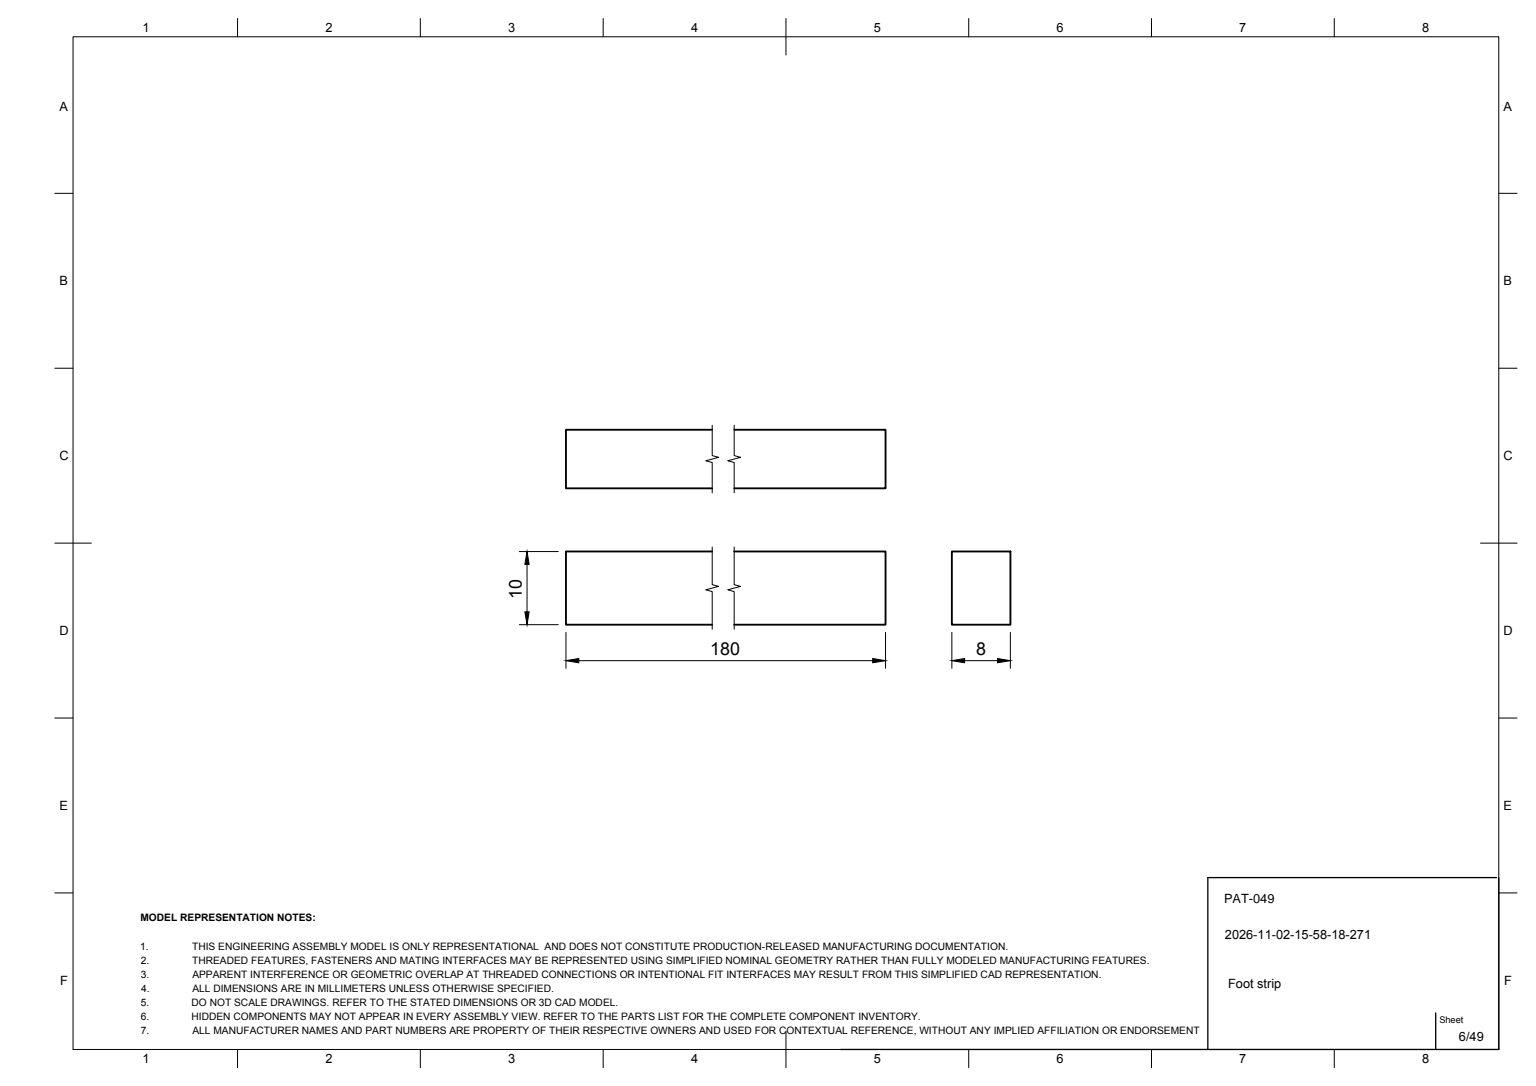
ISO-10303-21;
HEADER;
/* Generated by software containing ST-Developer
 * from STEP Tools, Inc. (www.steptools.com) 
 */

FILE_DESCRIPTION(
/* description */ ('Hand drill press frame (manual)'),
/* implementation_level */ '2;1');

FILE_NAME(
/* name */ 'Foot strip.step',
/* time_stamp */ '2026-10-28T03:25:28-07:00',
/* author */ (''),
/* organization */ (''),
/* preprocessor_version */ 'ST-DEVELOPER v20.2',
/* originating_system */ 'Autodesk Translation Framework v15.17.0.0',
/* authorisation */ '');

FILE_SCHEMA (('AUTOMOTIVE_DESIGN { 1 0 10303 214 3 1 1 }'));
ENDSEC;

DATA;
#10=MECHANICAL_DESIGN_GEOMETRIC_PRESENTATION_REPRESENTATION('',(#620),#33299);
#530=SHAPE_REPRESENTATION_RELATIONSHIP('SRR','None',#33489,#575);
#575=ADVANCED_BREP_SHAPE_REPRESENTATION('',(#672),#33251);
#620=STYLED_ITEM('',(#33800),#672);
#672=MANIFOLD_SOLID_BREP('Body1',#12638);
#893=PLANE('',#13216);
#894=PLANE('',#13217);
#895=PLANE('',#13218);
#896=PLANE('',#13219);
#897=PLANE('',#13220);
#898=PLANE('',#13221);
#1351=FACE_OUTER_BOUND('',#2052,.T.);
#1352=FACE_OUTER_BOUND('',#2053,.T.);
#1353=FACE_OUTER_BOUND('',#2054,.T.);
#1354=FACE_OUTER_BOUND('',#2055,.T.);
#1355=FACE_OUTER_BOUND('',#2056,.T.);
#1356=FACE_OUTER_BOUND('',#2057,.T.);
#2052=EDGE_LOOP('',(#8481,#8482,#8483,#8484));
#2053=EDGE_LOOP('',(#8485,#8486,#8487,#8488));
#2054=EDGE_LOOP('',(#8489,#8490,#8491,#8492));
#2055=EDGE_LOOP('',(#8493,#8494,#8495,#8496));
#2056=EDGE_LOOP('',(#8497,#8498,#8499,#8500));
#2057=EDGE_LOOP('',(#8501,#8502,#8503,#8504));
#2902=LINE('',#17959,#4067);
#2903=LINE('',#17961,#4068);
#2904=LINE('',#17963,#4069);
#2905=LINE('',#17964,#4070);
#2906=LINE('',#17967,#4071);
#2907=LINE('',#17969,#4072);
#2908=LINE('',#17970,#4073);
#2909=LINE('',#17973,#4074);
#2910=LINE('',#17975,#4075);
#2911=LINE('',#17976,#4076);
#2912=LINE('',#17978,#4077);
#2913=LINE('',#17979,#4078);
#4067=VECTOR('',#14443,1.);
#4068=VECTOR('',#14444,1.);
#4069=VECTOR('',#14445,1.);
#4070=VECTOR('',#14446,1.);
#4071=VECTOR('',#14449,1.);
#4072=VECTOR('',#14450,1.);
#4073=VECTOR('',#14451,1.);
#4074=VECTOR('',#14454,1.);
#4075=VECTOR('',#14455,1.);
#4076=VECTOR('',#14456,1.);
#4077=VECTOR('',#14459,1.);
#4078=VECTOR('',#14460,1.);
#5633=VERTEX_POINT('',#17957);
#5634=VERTEX_POINT('',#17958);
#5635=VERTEX_POINT('',#17960);
#5636=VERTEX_POINT('',#17962);
#5637=VERTEX_POINT('',#17966);
#5638=VERTEX_POINT('',#17968);
#5639=VERTEX_POINT('',#17972);
#5640=VERTEX_POINT('',#17974);
#6769=EDGE_CURVE('',#5633,#5634,#2902,.T.);
#6770=EDGE_CURVE('',#5634,#5635,#2903,.T.);
#6771=EDGE_CURVE('',#5636,#5635,#2904,.T.);
#6772=EDGE_CURVE('',#5633,#5636,#2905,.T.);
#6773=EDGE_CURVE('',#5637,#5633,#2906,.T.);
#6774=EDGE_CURVE('',#5638,#5636,#2907,.T.);
#6775=EDGE_CURVE('',#5637,#5638,#2908,.T.);
#6776=EDGE_CURVE('',#5639,#5637,#2909,.T.);
#6777=EDGE_CURVE('',#5640,#5638,#2910,.T.);
#6778=EDGE_CURVE('',#5639,#5640,#2911,.T.);
#6779=EDGE_CURVE('',#5634,#5639,#2912,.T.);
#6780=EDGE_CURVE('',#5635,#5640,#2913,.T.);
#8481=ORIENTED_EDGE('',*,*,#6769,.T.);
#8482=ORIENTED_EDGE('',*,*,#6770,.T.);
#8483=ORIENTED_EDGE('',*,*,#6771,.F.);
#8484=ORIENTED_EDGE('',*,*,#6772,.F.);
#8485=ORIENTED_EDGE('',*,*,#6773,.T.);
#8486=ORIENTED_EDGE('',*,*,#6772,.T.);
#8487=ORIENTED_EDGE('',*,*,#6774,.F.);
#8488=ORIENTED_EDGE('',*,*,#6775,.F.);
#8489=ORIENTED_EDGE('',*,*,#6776,.T.);
#8490=ORIENTED_EDGE('',*,*,#6775,.T.);
#8491=ORIENTED_EDGE('',*,*,#6777,.F.);
#8492=ORIENTED_EDGE('',*,*,#6778,.F.);
#8493=ORIENTED_EDGE('',*,*,#6779,.T.);
#8494=ORIENTED_EDGE('',*,*,#6778,.T.);
#8495=ORIENTED_EDGE('',*,*,#6780,.F.);
#8496=ORIENTED_EDGE('',*,*,#6770,.F.);
#8497=ORIENTED_EDGE('',*,*,#6780,.T.);
#8498=ORIENTED_EDGE('',*,*,#6777,.T.);
#8499=ORIENTED_EDGE('',*,*,#6774,.T.);
#8500=ORIENTED_EDGE('',*,*,#6771,.T.);
#8501=ORIENTED_EDGE('',*,*,#6779,.F.);
#8502=ORIENTED_EDGE('',*,*,#6769,.F.);
#8503=ORIENTED_EDGE('',*,*,#6773,.F.);
#8504=ORIENTED_EDGE('',*,*,#6776,.F.);
#11960=ADVANCED_FACE('',(#1351),#893,.T.);
#11961=ADVANCED_FACE('',(#1352),#894,.T.);
#11962=ADVANCED_FACE('',(#1353),#895,.T.);
#11963=ADVANCED_FACE('',(#1354),#896,.T.);
#11964=ADVANCED_FACE('',(#1355),#897,.T.);
#11965=ADVANCED_FACE('',(#1356),#898,.F.);
#12638=CLOSED_SHELL('',(#11960,#11961,#11962,#11963,#11964,#11965));
#13215=AXIS2_PLACEMENT_3D('',#17955,#14439,#14440);
#13216=AXIS2_PLACEMENT_3D('',#17956,#14441,#14442);
#13217=AXIS2_PLACEMENT_3D('',#17965,#14447,#14448);
#13218=AXIS2_PLACEMENT_3D('',#17971,#14452,#14453);
#13219=AXIS2_PLACEMENT_3D('',#17977,#14457,#14458);
#13220=AXIS2_PLACEMENT_3D('',#17980,#14461,#14462);
#13221=AXIS2_PLACEMENT_3D('',#17981,#14463,#14464);
#14439=DIRECTION('axis',(0.,0.,1.));
#14440=DIRECTION('refdir',(1.,0.,0.));
#14441=DIRECTION('center_axis',(0.,1.,0.));
#14442=DIRECTION('ref_axis',(-1.,0.,0.));
#14443=DIRECTION('',(-1.,0.,0.));
#14444=DIRECTION('',(0.,0.,1.));
#14445=DIRECTION('',(-1.,0.,0.));
#14446=DIRECTION('',(0.,0.,1.));
#14447=DIRECTION('center_axis',(1.,0.,0.));
#14448=DIRECTION('ref_axis',(0.,1.,0.));
#14449=DIRECTION('',(0.,1.,0.));
#14450=DIRECTION('',(0.,1.,0.));
#14451=DIRECTION('',(0.,0.,1.));
#14452=DIRECTION('center_axis',(0.,-1.,0.));
#14453=DIRECTION('ref_axis',(1.,0.,0.));
#14454=DIRECTION('',(1.,0.,0.));
#14455=DIRECTION('',(1.,0.,0.));
#14456=DIRECTION('',(0.,0.,1.));
#14457=DIRECTION('center_axis',(-1.,0.,0.));
#14458=DIRECTION('ref_axis',(0.,-1.,0.));
#14459=DIRECTION('',(0.,-1.,0.));
#14460=DIRECTION('',(0.,-1.,0.));
#14461=DIRECTION('center_axis',(0.,0.,1.));
#14462=DIRECTION('ref_axis',(1.,0.,0.));
#14463=DIRECTION('center_axis',(0.,0.,1.));
#14464=DIRECTION('ref_axis',(1.,0.,0.));
#17955=CARTESIAN_POINT('',(0.,0.,0.));
#17956=CARTESIAN_POINT('Origin',(-7.,9.,-0.8));
#17957=CARTESIAN_POINT('',(-7.,9.,-0.8));
#17958=CARTESIAN_POINT('',(-8.,9.,-0.8));
#17959=CARTESIAN_POINT('',(-7.,9.,-0.8));
#17960=CARTESIAN_POINT('',(-8.,9.,0.));
#17961=CARTESIAN_POINT('',(-8.,9.,-0.8));
#17962=CARTESIAN_POINT('',(-7.,9.,0.));
#17963=CARTESIAN_POINT('',(-7.,9.,0.));
#17964=CARTESIAN_POINT('',(-7.,9.,-0.8));
#17965=CARTESIAN_POINT('Origin',(-7.,-9.,-0.8));
#17966=CARTESIAN_POINT('',(-7.,-9.,-0.8));
#17967=CARTESIAN_POINT('',(-7.,-9.,-0.8));
#17968=CARTESIAN_POINT('',(-7.,-9.,0.));
#17969=CARTESIAN_POINT('',(-7.,-9.,0.));
#17970=CARTESIAN_POINT('',(-7.,-9.,-0.8));
#17971=CARTESIAN_POINT('Origin',(-8.,-9.,-0.8));
#17972=CARTESIAN_POINT('',(-8.,-9.,-0.8));
#17973=CARTESIAN_POINT('',(-8.,-9.,-0.8));
#17974=CARTESIAN_POINT('',(-8.,-9.,0.));
#17975=CARTESIAN_POINT('',(-8.,-9.,0.));
#17976=CARTESIAN_POINT('',(-8.,-9.,-0.8));
#17977=CARTESIAN_POINT('Origin',(-8.,9.,-0.8));
#17978=CARTESIAN_POINT('',(-8.,9.,-0.8));
#17979=CARTESIAN_POINT('',(-8.,9.,0.));
#17980=CARTESIAN_POINT('Origin',(-7.5,0.,0.));
#17981=CARTESIAN_POINT('Origin',(-7.5,0.,-0.8));
#33199=UNCERTAINTY_MEASURE_WITH_UNIT(LENGTH_MEASURE(0.001),#33300,
'DISTANCE_ACCURACY_VALUE',
'Maximum model space distance between geometric entities at asserted c
onnectivities');
#33247=UNCERTAINTY_MEASURE_WITH_UNIT(LENGTH_MEASURE(0.001),#33300,
'DISTANCE_ACCURACY_VALUE',
'Maximum model space distance between geometric entities at asserted c
onnectivities');
#33251=(
GEOMETRIC_REPRESENTATION_CONTEXT(3)
GLOBAL_UNCERTAINTY_ASSIGNED_CONTEXT((#33199))
GLOBAL_UNIT_ASSIGNED_CONTEXT((#33300,#33302,#33303))
REPRESENTATION_CONTEXT('','3D')
);
#33299=(
GEOMETRIC_REPRESENTATION_CONTEXT(3)
GLOBAL_UNCERTAINTY_ASSIGNED_CONTEXT((#33247))
GLOBAL_UNIT_ASSIGNED_CONTEXT((#33300,#33302,#33303))
REPRESENTATION_CONTEXT('','3D')
);
#33300=(
LENGTH_UNIT()
NAMED_UNIT(*)
SI_UNIT(.CENTI.,.METRE.)
);
#33302=(
NAMED_UNIT(*)
PLANE_ANGLE_UNIT()
SI_UNIT($,.RADIAN.)
);
#33303=(
NAMED_UNIT(*)
SI_UNIT($,.STERADIAN.)
SOLID_ANGLE_UNIT()
);
#33307=SHAPE_DEFINITION_REPRESENTATION(#33358,#33489);
#33358=PRODUCT_DEFINITION_SHAPE('',$,#33541);
#33489=SHAPE_REPRESENTATION('',(#13215),#33251);
#33537=PRODUCT_DEFINITION_CONTEXT('part definition',#33692,'design');
#33541=PRODUCT_DEFINITION('Foot strip','Foot strip',#33592,#33537);
#33592=PRODUCT_DEFINITION_FORMATION('',$,#33697);
#33692=APPLICATION_CONTEXT(
'Core Data for Automotive Mechanical Design Process');
#33693=PRODUCT_CONTEXT('part definition',#33692,'mechanical');
#33697=PRODUCT('Foot strip','Foot strip','Foot strip',(#33693));
#33794=COLOUR_RGB('Light Blue',0.38,0.62,0.78);
#33795=FILL_AREA_STYLE_COLOUR('',#33794);
#33796=FILL_AREA_STYLE('',(#33795));
#33797=SURFACE_STYLE_FILL_AREA(#33796);
#33798=SURFACE_SIDE_STYLE('',(#33797));
#33799=SURFACE_STYLE_USAGE(.BOTH.,#33798);
#33800=PRESENTATION_STYLE_ASSIGNMENT((#33799));
ENDSEC;
END-ISO-10303-21;
